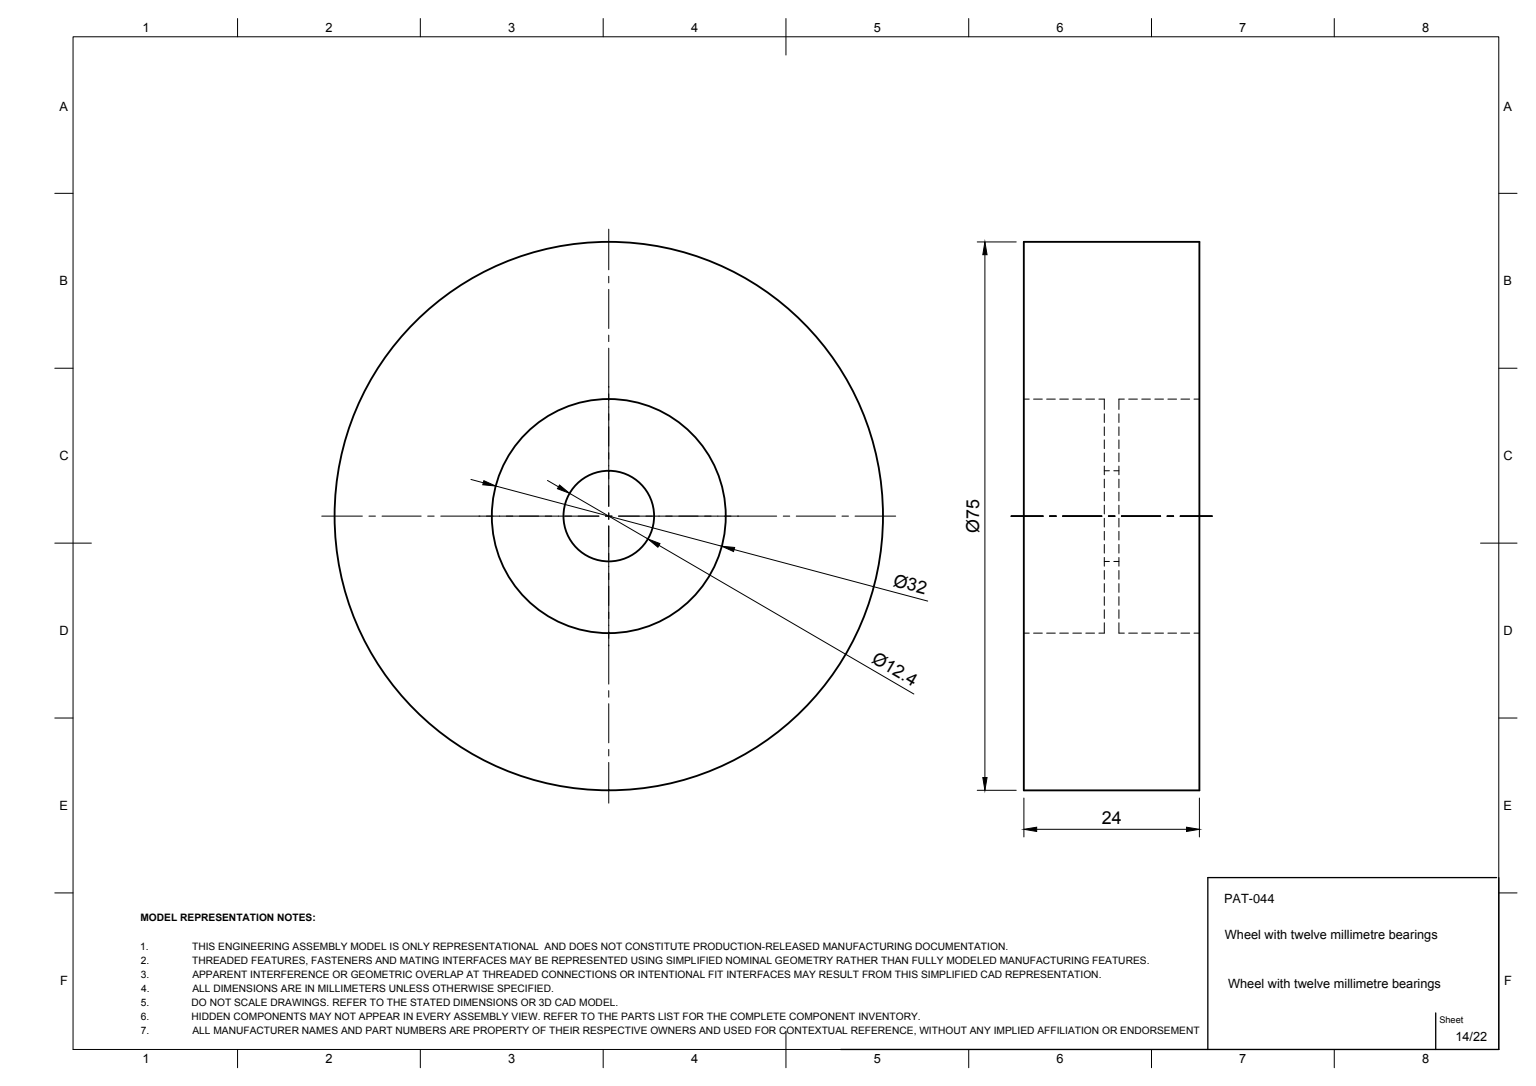
ISO-10303-21;
HEADER;
/* Generated by software containing ST-Developer
 * from STEP Tools, Inc. (www.steptools.com) 
 */

FILE_DESCRIPTION(
/* description */ ('Four-wheel beam trolley'),
/* implementation_level */ '2;1');

FILE_NAME(
/* name */ 'Wheel with twelve millimetre bearings.step',
/* time_stamp */ '2026-10-29T16:22:06-07:00',
/* author */ (''),
/* organization */ (''),
/* preprocessor_version */ 'ST-DEVELOPER v20.2',
/* originating_system */ 'Autodesk Translation Framework v15.17.0.0',
/* authorisation */ '');

FILE_SCHEMA (('AUTOMOTIVE_DESIGN { 1 0 10303 214 3 1 1 }'));
ENDSEC;

DATA;
#10=MECHANICAL_DESIGN_GEOMETRIC_PRESENTATION_REPRESENTATION('',(#288),#4777);
#254=SHAPE_REPRESENTATION_RELATIONSHIP('SRR','None',#4884,#271);
#271=ADVANCED_BREP_SHAPE_REPRESENTATION('',(#310),#4769);
#288=STYLED_ITEM('',(#5056),#310);
#310=MANIFOLD_SOLID_BREP('Body1',#2377);
#350=FACE_BOUND('',#704,.T.);
#351=FACE_BOUND('',#707,.T.);
#352=FACE_BOUND('',#711,.T.);
#353=FACE_BOUND('',#713,.T.);
#420=PLANE('',#2772);
#421=PLANE('',#2777);
#422=PLANE('',#2783);
#423=PLANE('',#2784);
#529=FACE_OUTER_BOUND('',#702,.T.);
#530=FACE_OUTER_BOUND('',#703,.T.);
#531=FACE_OUTER_BOUND('',#705,.T.);
#532=FACE_OUTER_BOUND('',#706,.T.);
#533=FACE_OUTER_BOUND('',#708,.T.);
#534=FACE_OUTER_BOUND('',#709,.T.);
#535=FACE_OUTER_BOUND('',#710,.T.);
#536=FACE_OUTER_BOUND('',#712,.T.);
#702=EDGE_LOOP('',(#1941,#1942,#1943,#1944));
#703=EDGE_LOOP('',(#1945));
#704=EDGE_LOOP('',(#1946));
#705=EDGE_LOOP('',(#1947,#1948,#1949,#1950));
#706=EDGE_LOOP('',(#1951));
#707=EDGE_LOOP('',(#1952));
#708=EDGE_LOOP('',(#1953,#1954,#1955,#1956));
#709=EDGE_LOOP('',(#1957,#1958,#1959,#1960));
#710=EDGE_LOOP('',(#1961));
#711=EDGE_LOOP('',(#1962));
#712=EDGE_LOOP('',(#1963));
#713=EDGE_LOOP('',(#1964));
#878=LINE('',#4159,#1001);
#879=LINE('',#4168,#1002);
#880=LINE('',#4174,#1003);
#881=LINE('',#4179,#1004);
#1001=VECTOR('',#3417,1.6);
#1002=VECTOR('',#3428,1.6);
#1003=VECTOR('',#3437,0.62);
#1004=VECTOR('',#3442,3.75);
#1080=CIRCLE('',#2770,1.6);
#1081=CIRCLE('',#2771,1.6);
#1082=CIRCLE('',#2773,0.62);
#1083=CIRCLE('',#2775,1.6);
#1084=CIRCLE('',#2776,1.6);
#1085=CIRCLE('',#2778,0.62);
#1086=CIRCLE('',#2781,3.75);
#1087=CIRCLE('',#2782,3.75);
#1264=VERTEX_POINT('',#4156);
#1265=VERTEX_POINT('',#4158);
#1266=VERTEX_POINT('',#4162);
#1267=VERTEX_POINT('',#4165);
#1268=VERTEX_POINT('',#4167);
#1269=VERTEX_POINT('',#4171);
#1270=VERTEX_POINT('',#4176);
#1271=VERTEX_POINT('',#4178);
#1508=EDGE_CURVE('',#1264,#1264,#1080,.T.);
#1509=EDGE_CURVE('',#1264,#1265,#878,.T.);
#1510=EDGE_CURVE('',#1265,#1265,#1081,.T.);
#1511=EDGE_CURVE('',#1266,#1266,#1082,.T.);
#1512=EDGE_CURVE('',#1267,#1267,#1083,.T.);
#1513=EDGE_CURVE('',#1267,#1268,#879,.T.);
#1514=EDGE_CURVE('',#1268,#1268,#1084,.T.);
#1515=EDGE_CURVE('',#1269,#1269,#1085,.T.);
#1516=EDGE_CURVE('',#1269,#1266,#880,.T.);
#1517=EDGE_CURVE('',#1270,#1270,#1086,.T.);
#1518=EDGE_CURVE('',#1270,#1271,#881,.T.);
#1519=EDGE_CURVE('',#1271,#1271,#1087,.T.);
#1941=ORIENTED_EDGE('',*,*,#1508,.F.);
#1942=ORIENTED_EDGE('',*,*,#1509,.T.);
#1943=ORIENTED_EDGE('',*,*,#1510,.F.);
#1944=ORIENTED_EDGE('',*,*,#1509,.F.);
#1945=ORIENTED_EDGE('',*,*,#1508,.T.);
#1946=ORIENTED_EDGE('',*,*,#1511,.F.);
#1947=ORIENTED_EDGE('',*,*,#1512,.F.);
#1948=ORIENTED_EDGE('',*,*,#1513,.T.);
#1949=ORIENTED_EDGE('',*,*,#1514,.T.);
#1950=ORIENTED_EDGE('',*,*,#1513,.F.);
#1951=ORIENTED_EDGE('',*,*,#1514,.F.);
#1952=ORIENTED_EDGE('',*,*,#1515,.F.);
#1953=ORIENTED_EDGE('',*,*,#1515,.T.);
#1954=ORIENTED_EDGE('',*,*,#1516,.T.);
#1955=ORIENTED_EDGE('',*,*,#1511,.T.);
#1956=ORIENTED_EDGE('',*,*,#1516,.F.);
#1957=ORIENTED_EDGE('',*,*,#1517,.F.);
#1958=ORIENTED_EDGE('',*,*,#1518,.T.);
#1959=ORIENTED_EDGE('',*,*,#1519,.T.);
#1960=ORIENTED_EDGE('',*,*,#1518,.F.);
#1961=ORIENTED_EDGE('',*,*,#1517,.T.);
#1962=ORIENTED_EDGE('',*,*,#1510,.T.);
#1963=ORIENTED_EDGE('',*,*,#1519,.F.);
#1964=ORIENTED_EDGE('',*,*,#1512,.T.);
#2200=CYLINDRICAL_SURFACE('',#2769,1.6);
#2201=CYLINDRICAL_SURFACE('',#2774,1.6);
#2202=CYLINDRICAL_SURFACE('',#2779,0.62);
#2203=CYLINDRICAL_SURFACE('',#2780,3.75);
#2305=ADVANCED_FACE('',(#529),#2200,.F.);
#2306=ADVANCED_FACE('',(#530,#350),#420,.T.);
#2307=ADVANCED_FACE('',(#531),#2201,.F.);
#2308=ADVANCED_FACE('',(#532,#351),#421,.F.);
#2309=ADVANCED_FACE('',(#533),#2202,.F.);
#2310=ADVANCED_FACE('',(#534),#2203,.T.);
#2311=ADVANCED_FACE('',(#535,#352),#422,.T.);
#2312=ADVANCED_FACE('',(#536,#353),#423,.F.);
#2377=CLOSED_SHELL('',(#2305,#2306,#2307,#2308,#2309,#2310,#2311,#2312));
#2768=AXIS2_PLACEMENT_3D('',#4154,#3411,#3412);
#2769=AXIS2_PLACEMENT_3D('',#4155,#3413,#3414);
#2770=AXIS2_PLACEMENT_3D('',#4157,#3415,#3416);
#2771=AXIS2_PLACEMENT_3D('',#4160,#3418,#3419);
#2772=AXIS2_PLACEMENT_3D('',#4161,#3420,#3421);
#2773=AXIS2_PLACEMENT_3D('',#4163,#3422,#3423);
#2774=AXIS2_PLACEMENT_3D('',#4164,#3424,#3425);
#2775=AXIS2_PLACEMENT_3D('',#4166,#3426,#3427);
#2776=AXIS2_PLACEMENT_3D('',#4169,#3429,#3430);
#2777=AXIS2_PLACEMENT_3D('',#4170,#3431,#3432);
#2778=AXIS2_PLACEMENT_3D('',#4172,#3433,#3434);
#2779=AXIS2_PLACEMENT_3D('',#4173,#3435,#3436);
#2780=AXIS2_PLACEMENT_3D('',#4175,#3438,#3439);
#2781=AXIS2_PLACEMENT_3D('',#4177,#3440,#3441);
#2782=AXIS2_PLACEMENT_3D('',#4180,#3443,#3444);
#2783=AXIS2_PLACEMENT_3D('',#4181,#3445,#3446);
#2784=AXIS2_PLACEMENT_3D('',#4182,#3447,#3448);
#3411=DIRECTION('axis',(0.,0.,1.));
#3412=DIRECTION('refdir',(1.,0.,0.));
#3413=DIRECTION('center_axis',(0.,1.,0.));
#3414=DIRECTION('ref_axis',(1.,0.,0.));
#3415=DIRECTION('center_axis',(0.,1.,0.));
#3416=DIRECTION('ref_axis',(1.,0.,0.));
#3417=DIRECTION('',(0.,1.,0.));
#3418=DIRECTION('center_axis',(0.,-1.,0.));
#3419=DIRECTION('ref_axis',(1.,0.,0.));
#3420=DIRECTION('center_axis',(0.,1.,0.));
#3421=DIRECTION('ref_axis',(1.,0.,0.));
#3422=DIRECTION('center_axis',(0.,1.,0.));
#3423=DIRECTION('ref_axis',(1.,0.,0.));
#3424=DIRECTION('center_axis',(0.,1.,0.));
#3425=DIRECTION('ref_axis',(1.,0.,0.));
#3426=DIRECTION('center_axis',(0.,1.,0.));
#3427=DIRECTION('ref_axis',(1.,0.,0.));
#3428=DIRECTION('',(0.,1.,0.));
#3429=DIRECTION('center_axis',(0.,1.,0.));
#3430=DIRECTION('ref_axis',(1.,0.,0.));
#3431=DIRECTION('center_axis',(0.,1.,0.));
#3432=DIRECTION('ref_axis',(1.,0.,0.));
#3433=DIRECTION('center_axis',(0.,-1.,0.));
#3434=DIRECTION('ref_axis',(1.,0.,0.));
#3435=DIRECTION('center_axis',(0.,1.,0.));
#3436=DIRECTION('ref_axis',(1.,0.,0.));
#3437=DIRECTION('',(0.,1.,0.));
#3438=DIRECTION('center_axis',(0.,1.,0.));
#3439=DIRECTION('ref_axis',(1.,0.,0.));
#3440=DIRECTION('center_axis',(0.,1.,0.));
#3441=DIRECTION('ref_axis',(1.,0.,0.));
#3442=DIRECTION('',(0.,-1.,0.));
#3443=DIRECTION('center_axis',(0.,1.,0.));
#3444=DIRECTION('ref_axis',(1.,0.,0.));
#3445=DIRECTION('center_axis',(0.,1.,0.));
#3446=DIRECTION('ref_axis',(1.,0.,0.));
#3447=DIRECTION('center_axis',(0.,1.,0.));
#3448=DIRECTION('ref_axis',(1.,0.,0.));
#4154=CARTESIAN_POINT('',(0.,0.,0.));
#4155=CARTESIAN_POINT('Origin',(0.,0.1,4.));
#4156=CARTESIAN_POINT('',(-1.6,0.1,4.));
#4157=CARTESIAN_POINT('Origin',(0.,0.1,4.));
#4158=CARTESIAN_POINT('',(-1.6,1.2,4.));
#4159=CARTESIAN_POINT('',(-1.6,0.1,4.));
#4160=CARTESIAN_POINT('Origin',(0.,1.2,4.));
#4161=CARTESIAN_POINT('Origin',(0.,0.1,4.));
#4162=CARTESIAN_POINT('',(-0.62,0.1,4.));
#4163=CARTESIAN_POINT('Origin',(0.,0.1,4.));
#4164=CARTESIAN_POINT('Origin',(0.,-1.3,4.));
#4165=CARTESIAN_POINT('',(-1.6,-1.2,4.));
#4166=CARTESIAN_POINT('Origin',(0.,-1.2,4.));
#4167=CARTESIAN_POINT('',(-1.6,-0.0999999999999999,4.));
#4168=CARTESIAN_POINT('',(-1.6,-1.3,4.));
#4169=CARTESIAN_POINT('Origin',(0.,-0.0999999999999999,4.));
#4170=CARTESIAN_POINT('Origin',(0.,-0.0999999999999999,4.));
#4171=CARTESIAN_POINT('',(-0.62,-0.0999999999999999,4.));
#4172=CARTESIAN_POINT('Origin',(0.,-0.0999999999999999,4.));
#4173=CARTESIAN_POINT('Origin',(0.,-1.3,4.));
#4174=CARTESIAN_POINT('',(-0.62,-1.3,4.));
#4175=CARTESIAN_POINT('Origin',(0.,-1.2,4.));
#4176=CARTESIAN_POINT('',(-3.75,1.2,4.));
#4177=CARTESIAN_POINT('Origin',(0.,1.2,4.));
#4178=CARTESIAN_POINT('',(-3.75,-1.2,4.));
#4179=CARTESIAN_POINT('',(-3.75,-1.2,4.));
#4180=CARTESIAN_POINT('Origin',(0.,-1.2,4.));
#4181=CARTESIAN_POINT('Origin',(0.,1.2,4.));
#4182=CARTESIAN_POINT('Origin',(0.,-1.2,4.));
#4747=UNCERTAINTY_MEASURE_WITH_UNIT(LENGTH_MEASURE(0.001),#4778,
'DISTANCE_ACCURACY_VALUE',
'Maximum model space distance between geometric entities at asserted c
onnectivities');
#4755=UNCERTAINTY_MEASURE_WITH_UNIT(LENGTH_MEASURE(0.001),#4778,
'DISTANCE_ACCURACY_VALUE',
'Maximum model space distance between geometric entities at asserted c
onnectivities');
#4769=(
GEOMETRIC_REPRESENTATION_CONTEXT(3)
GLOBAL_UNCERTAINTY_ASSIGNED_CONTEXT((#4747))
GLOBAL_UNIT_ASSIGNED_CONTEXT((#4778,#4780,#4781))
REPRESENTATION_CONTEXT('','3D')
);
#4777=(
GEOMETRIC_REPRESENTATION_CONTEXT(3)
GLOBAL_UNCERTAINTY_ASSIGNED_CONTEXT((#4755))
GLOBAL_UNIT_ASSIGNED_CONTEXT((#4778,#4780,#4781))
REPRESENTATION_CONTEXT('','3D')
);
#4778=(
LENGTH_UNIT()
NAMED_UNIT(*)
SI_UNIT(.CENTI.,.METRE.)
);
#4780=(
NAMED_UNIT(*)
PLANE_ANGLE_UNIT()
SI_UNIT($,.RADIAN.)
);
#4781=(
NAMED_UNIT(*)
SI_UNIT($,.STERADIAN.)
SOLID_ANGLE_UNIT()
);
#4795=SHAPE_DEFINITION_REPRESENTATION(#4848,#4884);
#4848=PRODUCT_DEFINITION_SHAPE('',$,#4906);
#4884=SHAPE_REPRESENTATION('',(#2768),#4769);
#4892=PRODUCT_DEFINITION_CONTEXT('part definition',#4957,'design');
#4906=PRODUCT_DEFINITION('Wheel with twelve millimetre bearings',
'Wheel with twelve millimetre bearings',#4927,#4892);
#4927=PRODUCT_DEFINITION_FORMATION('',$,#4972);
#4957=APPLICATION_CONTEXT(
'Core Data for Automotive Mechanical Design Process');
#4958=PRODUCT_CONTEXT('part definition',#4957,'mechanical');
#4972=PRODUCT('Wheel with twelve millimetre bearings',
'Wheel with twelve millimetre bearings',
'Wheel with twelve millimetre bearings',(#4958));
#5050=COLOUR_RGB('Grey',0.48,0.52,0.57);
#5051=FILL_AREA_STYLE_COLOUR('',#5050);
#5052=FILL_AREA_STYLE('',(#5051));
#5053=SURFACE_STYLE_FILL_AREA(#5052);
#5054=SURFACE_SIDE_STYLE('',(#5053));
#5055=SURFACE_STYLE_USAGE(.BOTH.,#5054);
#5056=PRESENTATION_STYLE_ASSIGNMENT((#5055));
ENDSEC;
END-ISO-10303-21;
